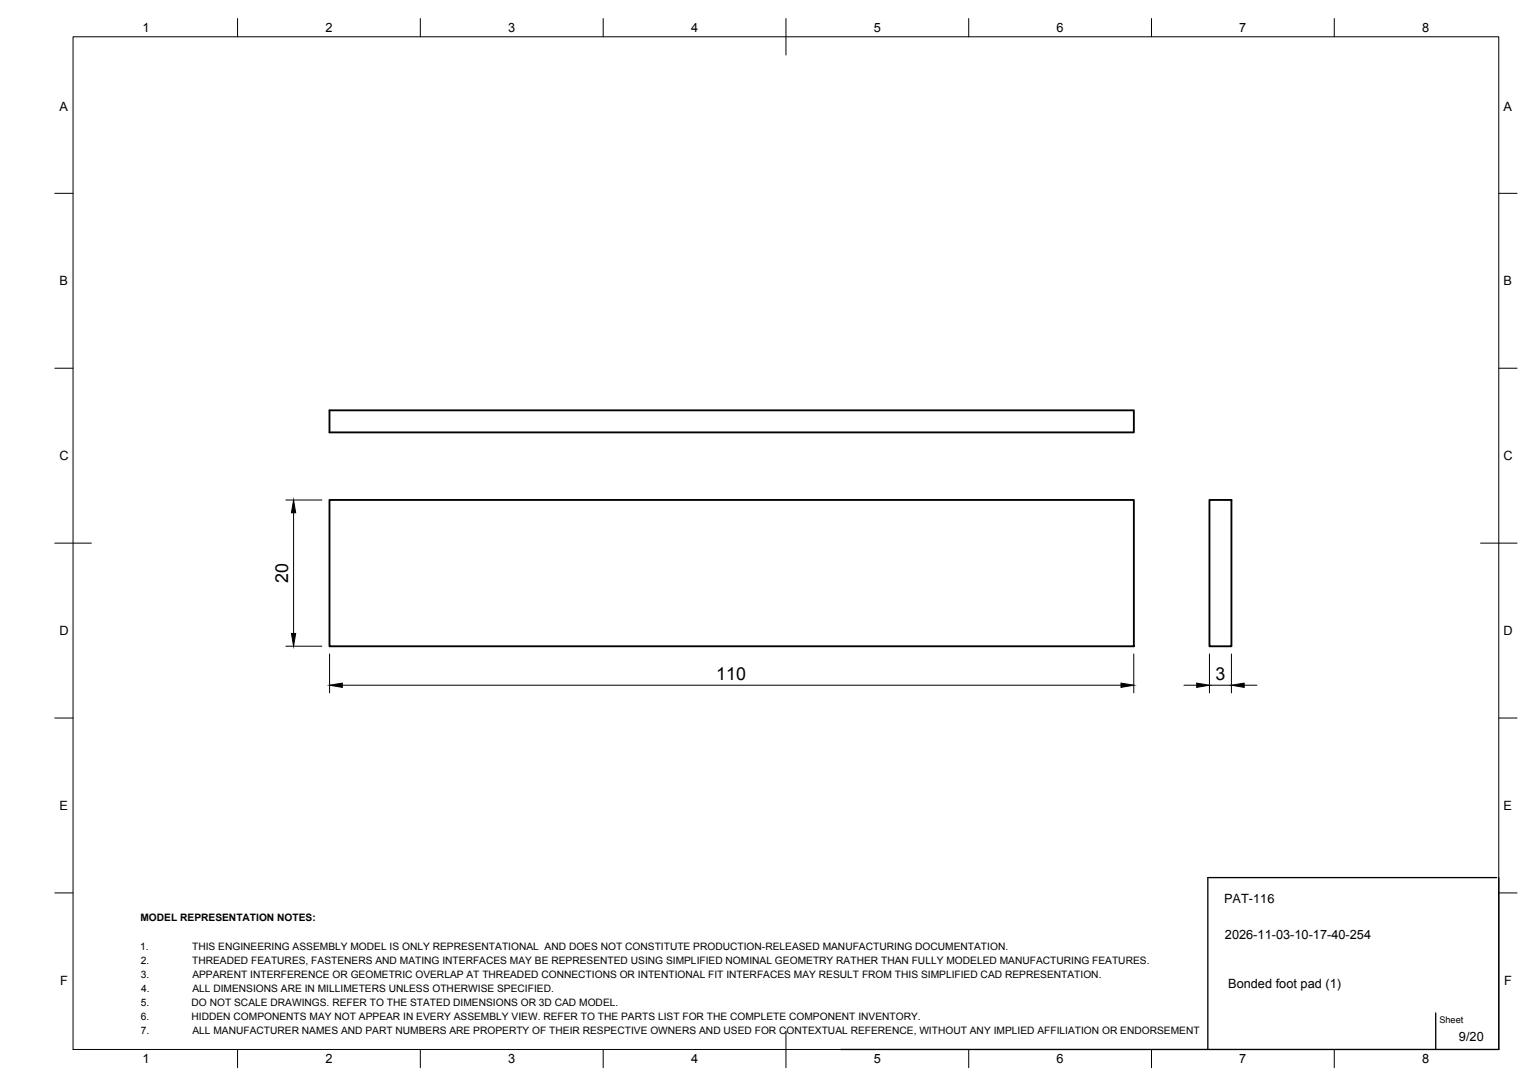
ISO-10303-21;
HEADER;
/* Generated by software containing ST-Developer
 * from STEP Tools, Inc. (www.steptools.com) 
 */

FILE_DESCRIPTION(
/* description */ ('V-block with clamp strap'),
/* implementation_level */ '2;1');

FILE_NAME(
/* name */ 'Bonded foot pad (1).step',
/* time_stamp */ '2026-10-27T10:50:53-07:00',
/* author */ (''),
/* organization */ (''),
/* preprocessor_version */ 'ST-DEVELOPER v20.2',
/* originating_system */ 'Autodesk Translation Framework v15.17.0.0',
/* authorisation */ '');

FILE_SCHEMA (('AUTOMOTIVE_DESIGN { 1 0 10303 214 3 1 1 }'));
ENDSEC;

DATA;
#10=MECHANICAL_DESIGN_GEOMETRIC_PRESENTATION_REPRESENTATION('',(#270),#7344);
#228=SHAPE_REPRESENTATION_RELATIONSHIP('SRR','None',#7446,#249);
#249=ADVANCED_BREP_SHAPE_REPRESENTATION('',(#291),#7325);
#270=STYLED_ITEM('',(#7624),#291);
#291=MANIFOLD_SOLID_BREP('Body1',#4152);
#612=FACE_OUTER_BOUND('',#886,.T.);
#613=FACE_OUTER_BOUND('',#887,.T.);
#614=FACE_OUTER_BOUND('',#888,.T.);
#615=FACE_OUTER_BOUND('',#889,.T.);
#616=FACE_OUTER_BOUND('',#890,.T.);
#617=FACE_OUTER_BOUND('',#891,.T.);
#886=EDGE_LOOP('',(#2936,#2937,#2938,#2939));
#887=EDGE_LOOP('',(#2940,#2941,#2942,#2943));
#888=EDGE_LOOP('',(#2944,#2945,#2946,#2947));
#889=EDGE_LOOP('',(#2948,#2949,#2950,#2951));
#890=EDGE_LOOP('',(#2952,#2953,#2954,#2955));
#891=EDGE_LOOP('',(#2956,#2957,#2958,#2959));
#1201=LINE('',#6346,#1566);
#1202=LINE('',#6348,#1567);
#1203=LINE('',#6350,#1568);
#1204=LINE('',#6351,#1569);
#1205=LINE('',#6354,#1570);
#1206=LINE('',#6356,#1571);
#1207=LINE('',#6357,#1572);
#1208=LINE('',#6360,#1573);
#1209=LINE('',#6362,#1574);
#1210=LINE('',#6363,#1575);
#1211=LINE('',#6365,#1576);
#1212=LINE('',#6366,#1577);
#1566=VECTOR('',#5111,1.);
#1567=VECTOR('',#5112,1.);
#1568=VECTOR('',#5113,1.);
#1569=VECTOR('',#5114,1.);
#1570=VECTOR('',#5117,1.);
#1571=VECTOR('',#5118,1.);
#1572=VECTOR('',#5119,1.);
#1573=VECTOR('',#5122,1.);
#1574=VECTOR('',#5123,1.);
#1575=VECTOR('',#5124,1.);
#1576=VECTOR('',#5127,1.);
#1577=VECTOR('',#5128,1.);
#1923=VERTEX_POINT('',#6344);
#1924=VERTEX_POINT('',#6345);
#1925=VERTEX_POINT('',#6347);
#1926=VERTEX_POINT('',#6349);
#1927=VERTEX_POINT('',#6353);
#1928=VERTEX_POINT('',#6355);
#1929=VERTEX_POINT('',#6359);
#1930=VERTEX_POINT('',#6361);
#2294=EDGE_CURVE('',#1923,#1924,#1201,.T.);
#2295=EDGE_CURVE('',#1924,#1925,#1202,.T.);
#2296=EDGE_CURVE('',#1926,#1925,#1203,.T.);
#2297=EDGE_CURVE('',#1923,#1926,#1204,.T.);
#2298=EDGE_CURVE('',#1927,#1923,#1205,.T.);
#2299=EDGE_CURVE('',#1928,#1926,#1206,.T.);
#2300=EDGE_CURVE('',#1927,#1928,#1207,.T.);
#2301=EDGE_CURVE('',#1929,#1927,#1208,.T.);
#2302=EDGE_CURVE('',#1930,#1928,#1209,.T.);
#2303=EDGE_CURVE('',#1929,#1930,#1210,.T.);
#2304=EDGE_CURVE('',#1924,#1929,#1211,.T.);
#2305=EDGE_CURVE('',#1925,#1930,#1212,.T.);
#2936=ORIENTED_EDGE('',*,*,#2294,.T.);
#2937=ORIENTED_EDGE('',*,*,#2295,.T.);
#2938=ORIENTED_EDGE('',*,*,#2296,.F.);
#2939=ORIENTED_EDGE('',*,*,#2297,.F.);
#2940=ORIENTED_EDGE('',*,*,#2298,.T.);
#2941=ORIENTED_EDGE('',*,*,#2297,.T.);
#2942=ORIENTED_EDGE('',*,*,#2299,.F.);
#2943=ORIENTED_EDGE('',*,*,#2300,.F.);
#2944=ORIENTED_EDGE('',*,*,#2301,.T.);
#2945=ORIENTED_EDGE('',*,*,#2300,.T.);
#2946=ORIENTED_EDGE('',*,*,#2302,.F.);
#2947=ORIENTED_EDGE('',*,*,#2303,.F.);
#2948=ORIENTED_EDGE('',*,*,#2304,.T.);
#2949=ORIENTED_EDGE('',*,*,#2303,.T.);
#2950=ORIENTED_EDGE('',*,*,#2305,.F.);
#2951=ORIENTED_EDGE('',*,*,#2295,.F.);
#2952=ORIENTED_EDGE('',*,*,#2305,.T.);
#2953=ORIENTED_EDGE('',*,*,#2302,.T.);
#2954=ORIENTED_EDGE('',*,*,#2299,.T.);
#2955=ORIENTED_EDGE('',*,*,#2296,.T.);
#2956=ORIENTED_EDGE('',*,*,#2304,.F.);
#2957=ORIENTED_EDGE('',*,*,#2294,.F.);
#2958=ORIENTED_EDGE('',*,*,#2298,.F.);
#2959=ORIENTED_EDGE('',*,*,#2301,.F.);
#3774=PLANE('',#4493);
#3775=PLANE('',#4494);
#3776=PLANE('',#4495);
#3777=PLANE('',#4496);
#3778=PLANE('',#4497);
#3779=PLANE('',#4498);
#3958=ADVANCED_FACE('',(#612),#3774,.T.);
#3959=ADVANCED_FACE('',(#613),#3775,.T.);
#3960=ADVANCED_FACE('',(#614),#3776,.T.);
#3961=ADVANCED_FACE('',(#615),#3777,.T.);
#3962=ADVANCED_FACE('',(#616),#3778,.T.);
#3963=ADVANCED_FACE('',(#617),#3779,.F.);
#4152=CLOSED_SHELL('',(#3958,#3959,#3960,#3961,#3962,#3963));
#4492=AXIS2_PLACEMENT_3D('',#6342,#5107,#5108);
#4493=AXIS2_PLACEMENT_3D('',#6343,#5109,#5110);
#4494=AXIS2_PLACEMENT_3D('',#6352,#5115,#5116);
#4495=AXIS2_PLACEMENT_3D('',#6358,#5120,#5121);
#4496=AXIS2_PLACEMENT_3D('',#6364,#5125,#5126);
#4497=AXIS2_PLACEMENT_3D('',#6367,#5129,#5130);
#4498=AXIS2_PLACEMENT_3D('',#6368,#5131,#5132);
#5107=DIRECTION('axis',(0.,0.,1.));
#5108=DIRECTION('refdir',(1.,0.,0.));
#5109=DIRECTION('center_axis',(0.,1.,0.));
#5110=DIRECTION('ref_axis',(-1.,0.,0.));
#5111=DIRECTION('',(-1.,0.,0.));
#5112=DIRECTION('',(0.,0.,1.));
#5113=DIRECTION('',(-1.,0.,0.));
#5114=DIRECTION('',(0.,0.,1.));
#5115=DIRECTION('center_axis',(1.,0.,0.));
#5116=DIRECTION('ref_axis',(0.,1.,0.));
#5117=DIRECTION('',(0.,1.,0.));
#5118=DIRECTION('',(0.,1.,0.));
#5119=DIRECTION('',(0.,0.,1.));
#5120=DIRECTION('center_axis',(0.,-1.,0.));
#5121=DIRECTION('ref_axis',(1.,0.,0.));
#5122=DIRECTION('',(1.,0.,0.));
#5123=DIRECTION('',(1.,0.,0.));
#5124=DIRECTION('',(0.,0.,1.));
#5125=DIRECTION('center_axis',(-1.,0.,0.));
#5126=DIRECTION('ref_axis',(0.,-1.,0.));
#5127=DIRECTION('',(0.,-1.,0.));
#5128=DIRECTION('',(0.,-1.,0.));
#5129=DIRECTION('center_axis',(0.,0.,1.));
#5130=DIRECTION('ref_axis',(1.,0.,0.));
#5131=DIRECTION('center_axis',(0.,0.,1.));
#5132=DIRECTION('ref_axis',(1.,0.,0.));
#6342=CARTESIAN_POINT('',(0.,0.,0.));
#6343=CARTESIAN_POINT('Origin',(18.,5.5,-1.3));
#6344=CARTESIAN_POINT('',(18.,5.5,-1.3));
#6345=CARTESIAN_POINT('',(16.,5.5,-1.3));
#6346=CARTESIAN_POINT('',(18.,5.5,-1.3));
#6347=CARTESIAN_POINT('',(16.,5.5,-1.));
#6348=CARTESIAN_POINT('',(16.,5.5,-1.3));
#6349=CARTESIAN_POINT('',(18.,5.5,-1.));
#6350=CARTESIAN_POINT('',(18.,5.5,-1.));
#6351=CARTESIAN_POINT('',(18.,5.5,-1.3));
#6352=CARTESIAN_POINT('Origin',(18.,-5.5,-1.3));
#6353=CARTESIAN_POINT('',(18.,-5.5,-1.3));
#6354=CARTESIAN_POINT('',(18.,-5.5,-1.3));
#6355=CARTESIAN_POINT('',(18.,-5.5,-1.));
#6356=CARTESIAN_POINT('',(18.,-5.5,-1.));
#6357=CARTESIAN_POINT('',(18.,-5.5,-1.3));
#6358=CARTESIAN_POINT('Origin',(16.,-5.5,-1.3));
#6359=CARTESIAN_POINT('',(16.,-5.5,-1.3));
#6360=CARTESIAN_POINT('',(16.,-5.5,-1.3));
#6361=CARTESIAN_POINT('',(16.,-5.5,-1.));
#6362=CARTESIAN_POINT('',(16.,-5.5,-1.));
#6363=CARTESIAN_POINT('',(16.,-5.5,-1.3));
#6364=CARTESIAN_POINT('Origin',(16.,5.5,-1.3));
#6365=CARTESIAN_POINT('',(16.,5.5,-1.3));
#6366=CARTESIAN_POINT('',(16.,5.5,-1.));
#6367=CARTESIAN_POINT('Origin',(17.,0.,-1.));
#6368=CARTESIAN_POINT('Origin',(17.,0.,-1.3));
#7299=UNCERTAINTY_MEASURE_WITH_UNIT(LENGTH_MEASURE(0.001),#7345,
'DISTANCE_ACCURACY_VALUE',
'Maximum model space distance between geometric entities at asserted c
onnectivities');
#7318=UNCERTAINTY_MEASURE_WITH_UNIT(LENGTH_MEASURE(0.001),#7345,
'DISTANCE_ACCURACY_VALUE',
'Maximum model space distance between geometric entities at asserted c
onnectivities');
#7325=(
GEOMETRIC_REPRESENTATION_CONTEXT(3)
GLOBAL_UNCERTAINTY_ASSIGNED_CONTEXT((#7299))
GLOBAL_UNIT_ASSIGNED_CONTEXT((#7345,#7347,#7348))
REPRESENTATION_CONTEXT('','3D')
);
#7344=(
GEOMETRIC_REPRESENTATION_CONTEXT(3)
GLOBAL_UNCERTAINTY_ASSIGNED_CONTEXT((#7318))
GLOBAL_UNIT_ASSIGNED_CONTEXT((#7345,#7347,#7348))
REPRESENTATION_CONTEXT('','3D')
);
#7345=(
LENGTH_UNIT()
NAMED_UNIT(*)
SI_UNIT(.CENTI.,.METRE.)
);
#7347=(
NAMED_UNIT(*)
PLANE_ANGLE_UNIT()
SI_UNIT($,.RADIAN.)
);
#7348=(
NAMED_UNIT(*)
SI_UNIT($,.STERADIAN.)
SOLID_ANGLE_UNIT()
);
#7355=SHAPE_DEFINITION_REPRESENTATION(#7380,#7446);
#7380=PRODUCT_DEFINITION_SHAPE('',$,#7472);
#7446=SHAPE_REPRESENTATION('',(#4492),#7325);
#7465=PRODUCT_DEFINITION_CONTEXT('part definition',#7542,'design');
#7472=PRODUCT_DEFINITION('Bonded foot pad (1)','Bonded foot pad (1)',#7497,
#7465);
#7497=PRODUCT_DEFINITION_FORMATION('',$,#7550);
#7542=APPLICATION_CONTEXT(
'Core Data for Automotive Mechanical Design Process');
#7543=PRODUCT_CONTEXT('part definition',#7542,'mechanical');
#7550=PRODUCT('Bonded foot pad (1)','Bonded foot pad (1)',
'Bonded foot pad (1)',(#7543));
#7618=COLOUR_RGB('Sky Blue',0.24,0.69,0.87);
#7619=FILL_AREA_STYLE_COLOUR('',#7618);
#7620=FILL_AREA_STYLE('',(#7619));
#7621=SURFACE_STYLE_FILL_AREA(#7620);
#7622=SURFACE_SIDE_STYLE('',(#7621));
#7623=SURFACE_STYLE_USAGE(.BOTH.,#7622);
#7624=PRESENTATION_STYLE_ASSIGNMENT((#7623));
ENDSEC;
END-ISO-10303-21;
